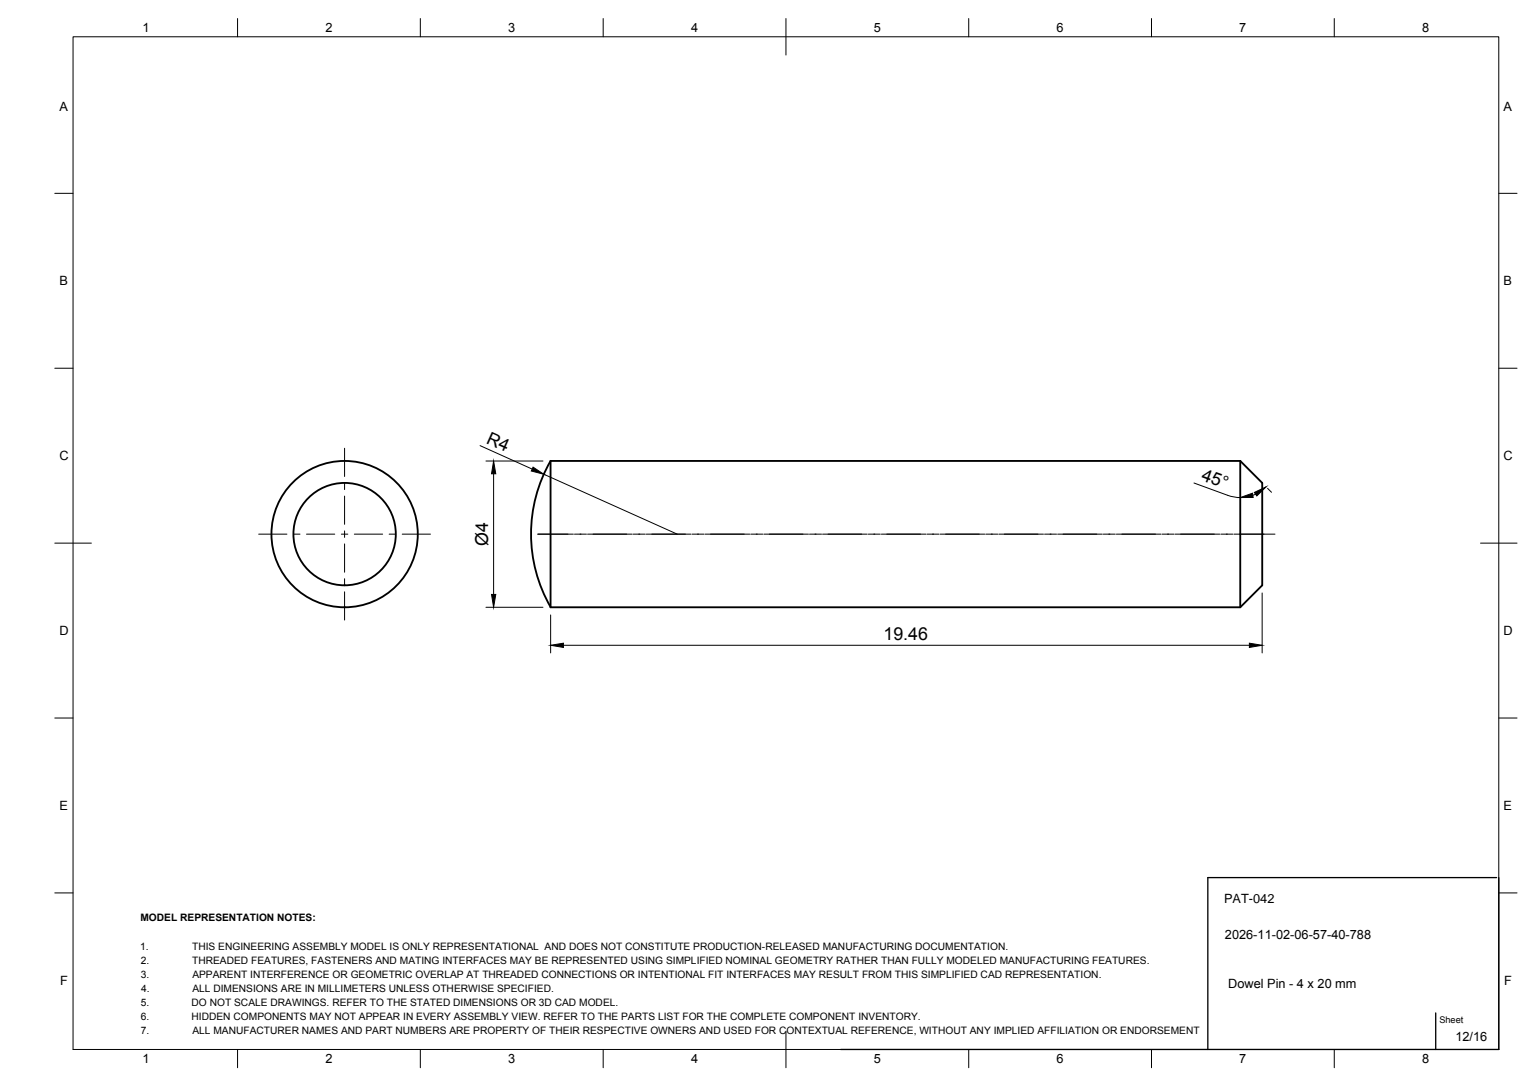
ISO-10303-21;
HEADER;
/* Generated by software containing ST-Developer
 * from STEP Tools, Inc. (www.steptools.com) 
 */

FILE_DESCRIPTION(
/* description */ ('Manifold and mounting hardware'),
/* implementation_level */ '2;1');

FILE_NAME(
/* name */ 'Dowel Pin - 4 x 20 mm.step',
/* time_stamp */ '2026-10-28T21:46:49-07:00',
/* author */ (''),
/* organization */ (''),
/* preprocessor_version */ 'ST-DEVELOPER v20.2',
/* originating_system */ 'Autodesk Translation Framework v15.17.0.0',
/* authorisation */ '');

FILE_SCHEMA (('AUTOMOTIVE_DESIGN { 1 0 10303 214 3 1 1 }'));
ENDSEC;

DATA;
#10=MECHANICAL_DESIGN_GEOMETRIC_PRESENTATION_REPRESENTATION('',(#161),#5638);
#17=SPHERICAL_SURFACE('',#3616,0.399999999999996);
#119=CONICAL_SURFACE('',#3620,0.17,0.785398163397449);
#133=SHAPE_REPRESENTATION_RELATIONSHIP('SRR','None',#5713,#147);
#147=ADVANCED_BREP_SHAPE_REPRESENTATION('',(#175),#5635);
#161=STYLED_ITEM('',(#5860),#175);
#175=MANIFOLD_SOLID_BREP('Body1',#3151);
#326=CYLINDRICAL_SURFACE('',#3618,0.2);
#496=FACE_OUTER_BOUND('',#754,.T.);
#497=FACE_OUTER_BOUND('',#755,.T.);
#498=FACE_OUTER_BOUND('',#756,.T.);
#499=FACE_OUTER_BOUND('',#757,.T.);
#754=EDGE_LOOP('',(#2758));
#755=EDGE_LOOP('',(#2759,#2760,#2761,#2762));
#756=EDGE_LOOP('',(#2763,#2764,#2765,#2766));
#757=EDGE_LOOP('',(#2767));
#886=CIRCLE('',#3617,0.2);
#887=CIRCLE('',#3619,0.2);
#888=CIRCLE('',#3621,0.14);
#1125=LINE('',#5495,#1372);
#1126=LINE('',#5499,#1373);
#1372=VECTOR('',#4522,0.2);
#1373=VECTOR('',#4527,0.17);
#1628=VERTEX_POINT('',#5490);
#1629=VERTEX_POINT('',#5493);
#1630=VERTEX_POINT('',#5497);
#2008=EDGE_CURVE('',#1628,#1628,#886,.T.);
#2009=EDGE_CURVE('',#1629,#1629,#887,.T.);
#2010=EDGE_CURVE('',#1629,#1628,#1125,.T.);
#2011=EDGE_CURVE('',#1630,#1630,#888,.T.);
#2012=EDGE_CURVE('',#1630,#1629,#1126,.T.);
#2758=ORIENTED_EDGE('',*,*,#2008,.F.);
#2759=ORIENTED_EDGE('',*,*,#2009,.F.);
#2760=ORIENTED_EDGE('',*,*,#2010,.T.);
#2761=ORIENTED_EDGE('',*,*,#2008,.T.);
#2762=ORIENTED_EDGE('',*,*,#2010,.F.);
#2763=ORIENTED_EDGE('',*,*,#2011,.F.);
#2764=ORIENTED_EDGE('',*,*,#2012,.T.);
#2765=ORIENTED_EDGE('',*,*,#2009,.T.);
#2766=ORIENTED_EDGE('',*,*,#2012,.F.);
#2767=ORIENTED_EDGE('',*,*,#2011,.T.);
#2942=PLANE('',#3622);
#3120=ADVANCED_FACE('',(#496),#17,.T.);
#3121=ADVANCED_FACE('',(#497),#326,.T.);
#3122=ADVANCED_FACE('',(#498),#119,.T.);
#3123=ADVANCED_FACE('',(#499),#2942,.T.);
#3151=CLOSED_SHELL('',(#3120,#3121,#3122,#3123));
#3615=AXIS2_PLACEMENT_3D('',#5488,#4512,#4513);
#3616=AXIS2_PLACEMENT_3D('',#5489,#4514,#4515);
#3617=AXIS2_PLACEMENT_3D('',#5491,#4516,#4517);
#3618=AXIS2_PLACEMENT_3D('',#5492,#4518,#4519);
#3619=AXIS2_PLACEMENT_3D('',#5494,#4520,#4521);
#3620=AXIS2_PLACEMENT_3D('',#5496,#4523,#4524);
#3621=AXIS2_PLACEMENT_3D('',#5498,#4525,#4526);
#3622=AXIS2_PLACEMENT_3D('',#5500,#4528,#4529);
#4512=DIRECTION('axis',(0.,0.,1.));
#4513=DIRECTION('refdir',(1.,0.,0.));
#4514=DIRECTION('center_axis',(6.12323399573679E-17,0.,1.));
#4515=DIRECTION('ref_axis',(1.,0.,0.));
#4516=DIRECTION('center_axis',(0.,-1.,0.));
#4517=DIRECTION('ref_axis',(1.,0.,0.));
#4518=DIRECTION('center_axis',(0.,-1.,0.));
#4519=DIRECTION('ref_axis',(1.,0.,0.));
#4520=DIRECTION('center_axis',(0.,-1.,0.));
#4521=DIRECTION('ref_axis',(1.,0.,0.));
#4522=DIRECTION('',(0.,1.,0.));
#4523=DIRECTION('center_axis',(0.,1.,0.));
#4524=DIRECTION('ref_axis',(1.,0.,0.));
#4525=DIRECTION('center_axis',(0.,-1.,0.));
#4526=DIRECTION('ref_axis',(1.,0.,0.));
#4527=DIRECTION('',(-0.707106781186548,0.707106781186547,-8.65956056235493E-17));
#4528=DIRECTION('center_axis',(0.,-1.,0.));
#4529=DIRECTION('ref_axis',(0.,0.,-1.));
#5488=CARTESIAN_POINT('',(0.,0.,0.));
#5489=CARTESIAN_POINT('Origin',(1.42247325030098E-15,1.60000000000001,0.));
#5490=CARTESIAN_POINT('',(-0.2,1.94641016151378,-2.44929359829471E-17));
#5491=CARTESIAN_POINT('Origin',(0.,1.94641016151378,0.));
#5492=CARTESIAN_POINT('Origin',(0.,1.00320508075689,0.));
#5493=CARTESIAN_POINT('',(-0.2,0.0600000000000001,-2.44929359829471E-17));
#5494=CARTESIAN_POINT('Origin',(0.,0.06,0.));
#5495=CARTESIAN_POINT('',(-0.2,1.00320508075689,-2.44929359829471E-17));
#5496=CARTESIAN_POINT('Origin',(0.,0.03,0.));
#5497=CARTESIAN_POINT('',(-0.14,3.46944695195361E-18,-1.71450551880629E-17));
#5498=CARTESIAN_POINT('Origin',(0.,0.,0.));
#5499=CARTESIAN_POINT('',(-0.17,0.03,-2.0818995585505E-17));
#5500=CARTESIAN_POINT('Origin',(0.,0.,0.));
#5618=UNCERTAINTY_MEASURE_WITH_UNIT(LENGTH_MEASURE(0.001),#5639,
'DISTANCE_ACCURACY_VALUE',
'Maximum model space distance between geometric entities at asserted c
onnectivities');
#5621=UNCERTAINTY_MEASURE_WITH_UNIT(LENGTH_MEASURE(0.001),#5639,
'DISTANCE_ACCURACY_VALUE',
'Maximum model space distance between geometric entities at asserted c
onnectivities');
#5635=(
GEOMETRIC_REPRESENTATION_CONTEXT(3)
GLOBAL_UNCERTAINTY_ASSIGNED_CONTEXT((#5618))
GLOBAL_UNIT_ASSIGNED_CONTEXT((#5639,#5641,#5642))
REPRESENTATION_CONTEXT('','3D')
);
#5638=(
GEOMETRIC_REPRESENTATION_CONTEXT(3)
GLOBAL_UNCERTAINTY_ASSIGNED_CONTEXT((#5621))
GLOBAL_UNIT_ASSIGNED_CONTEXT((#5639,#5641,#5642))
REPRESENTATION_CONTEXT('','3D')
);
#5639=(
LENGTH_UNIT()
NAMED_UNIT(*)
SI_UNIT(.CENTI.,.METRE.)
);
#5641=(
NAMED_UNIT(*)
PLANE_ANGLE_UNIT()
SI_UNIT($,.RADIAN.)
);
#5642=(
NAMED_UNIT(*)
SI_UNIT($,.STERADIAN.)
SOLID_ANGLE_UNIT()
);
#5656=SHAPE_DEFINITION_REPRESENTATION(#5674,#5713);
#5674=PRODUCT_DEFINITION_SHAPE('',$,#5730);
#5713=SHAPE_REPRESENTATION('',(#3615),#5635);
#5716=PRODUCT_DEFINITION_CONTEXT('part definition',#5766,'design');
#5730=PRODUCT_DEFINITION('Dowel Pin - 4 x 20 mm',
'Dowel Pin - 4 x 20 mm',#5746,#5716);
#5746=PRODUCT_DEFINITION_FORMATION('',$,#5781);
#5766=APPLICATION_CONTEXT(
'Core Data for Automotive Mechanical Design Process');
#5767=PRODUCT_CONTEXT('part definition',#5766,'mechanical');
#5781=PRODUCT('Dowel Pin - 4 x 20 mm','Dowel Pin - 4 x 20 mm',
'Dowel Pin - 4 x 20 mm',(#5767));
#5854=COLOUR_RGB('Grey',0.48,0.52,0.57);
#5855=FILL_AREA_STYLE_COLOUR('',#5854);
#5856=FILL_AREA_STYLE('',(#5855));
#5857=SURFACE_STYLE_FILL_AREA(#5856);
#5858=SURFACE_SIDE_STYLE('',(#5857));
#5859=SURFACE_STYLE_USAGE(.BOTH.,#5858);
#5860=PRESENTATION_STYLE_ASSIGNMENT((#5859));
ENDSEC;
END-ISO-10303-21;
